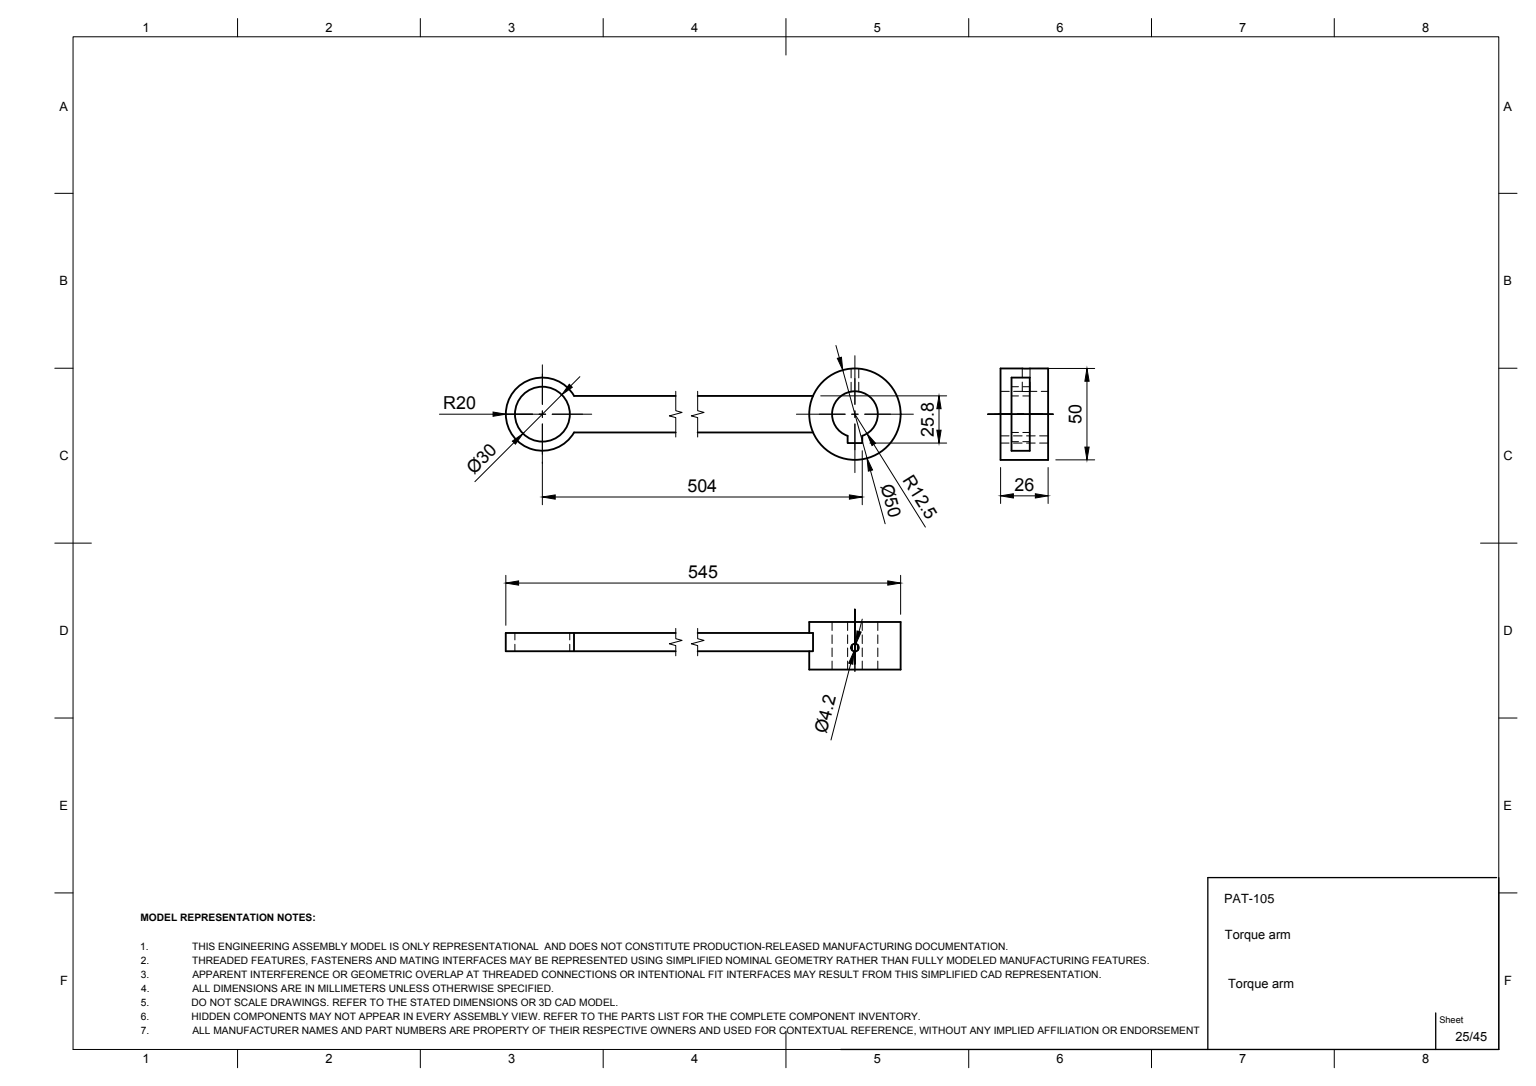
ISO-10303-21;
HEADER;
/* Generated by software containing ST-Developer
 * from STEP Tools, Inc. (www.steptools.com) 
 */

FILE_DESCRIPTION(
/* description */ ('Torque wrench calibration arm'),
/* implementation_level */ '2;1');

FILE_NAME(
/* name */ 'Torque arm.step',
/* time_stamp */ '2026-10-28T03:24:52-07:00',
/* author */ (''),
/* organization */ (''),
/* preprocessor_version */ 'ST-DEVELOPER v20.2',
/* originating_system */ 'Autodesk Translation Framework v15.17.0.0',
/* authorisation */ '');

FILE_SCHEMA (('AUTOMOTIVE_DESIGN { 1 0 10303 214 3 1 1 }'));
ENDSEC;

DATA;
#10=MECHANICAL_DESIGN_GEOMETRIC_PRESENTATION_REPRESENTATION('',(#453),#12783);
#271=B_SPLINE_CURVE_WITH_KNOTS('',3,(#11550,#11551,#11552,#11553,#11554,
#11555,#11556,#11557,#11558,#11559,#11560,#11561,#11562,#11563),
 .UNSPECIFIED.,.F.,.F.,(4,2,2,2,2,2,4),(0.779149138325153,0.792661737650616,
0.871926599437981,0.951191461225347,1.03045632301271,1.10972118480008,1.12323378412554),
 .UNSPECIFIED.);
#272=B_SPLINE_CURVE_WITH_KNOTS('',3,(#11569,#11570,#11571,#11572,#11573,
#11574,#11575,#11576,#11577,#11578,#11579,#11580,#11581,#11582,#11583,#11584,
#11585,#11586),.UNSPECIFIED.,.F.,.F.,(4,2,2,2,2,2,2,2,4),(0.,0.0791442954208927,
0.158288590841785,0.23743275251224,0.316576914182695,0.39572107585315,0.474865237523604,
0.554009532944497,0.63315382836539),.UNSPECIFIED.);
#273=B_SPLINE_CURVE_WITH_KNOTS('',3,(#11587,#11588,#11589,#11590,#11591,
#11592,#11593,#11594,#11595,#11596,#11597,#11598,#11599,#11600,#11601,#11602,
#11603,#11604),.UNSPECIFIED.,.F.,.F.,(4,2,2,2,2,2,2,2,4),(0.63315382836539,
0.712298123786282,0.791442419207175,0.87058658087763,0.949730742548085,
1.02887490421854,1.10801906588899,1.18716336130989,1.26630765673078),
 .UNSPECIFIED.);
#274=B_SPLINE_CURVE_WITH_KNOTS('',3,(#11607,#11608,#11609,#11610,#11611,
#11612,#11613,#11614,#11615,#11616,#11617,#11618,#11619,#11620),
 .UNSPECIFIED.,.F.,.F.,(4,2,2,2,2,2,4),(0.145021497508257,0.158534096833718,
0.237798958621084,0.317063820408449,0.396328682195814,0.47559354398318,
0.489106143308642),.UNSPECIFIED.);
#370=SHAPE_REPRESENTATION_RELATIONSHIP('SRR','None',#12953,#407);
#407=ADVANCED_BREP_SHAPE_REPRESENTATION('',(#505),#12762);
#453=STYLED_ITEM('',(#13205),#505);
#505=MANIFOLD_SOLID_BREP('Body1',#6524);
#608=FACE_BOUND('',#1588,.T.);
#609=FACE_BOUND('',#1590,.T.);
#610=FACE_BOUND('',#1594,.T.);
#611=FACE_BOUND('',#1597,.T.);
#612=FACE_BOUND('',#1600,.T.);
#613=FACE_BOUND('',#1601,.T.);
#614=FACE_BOUND('',#1603,.T.);
#785=PLANE('',#7454);
#786=PLANE('',#7459);
#787=PLANE('',#7460);
#788=PLANE('',#7461);
#789=PLANE('',#7462);
#790=PLANE('',#7463);
#791=PLANE('',#7474);
#792=PLANE('',#7476);
#793=PLANE('',#7477);
#794=PLANE('',#7479);
#795=PLANE('',#7482);
#1109=FACE_OUTER_BOUND('',#1581,.T.);
#1110=FACE_OUTER_BOUND('',#1582,.T.);
#1111=FACE_OUTER_BOUND('',#1583,.T.);
#1112=FACE_OUTER_BOUND('',#1584,.T.);
#1113=FACE_OUTER_BOUND('',#1585,.T.);
#1114=FACE_OUTER_BOUND('',#1586,.T.);
#1115=FACE_OUTER_BOUND('',#1587,.T.);
#1116=FACE_OUTER_BOUND('',#1589,.T.);
#1117=FACE_OUTER_BOUND('',#1591,.T.);
#1118=FACE_OUTER_BOUND('',#1592,.T.);
#1119=FACE_OUTER_BOUND('',#1593,.T.);
#1120=FACE_OUTER_BOUND('',#1595,.T.);
#1121=FACE_OUTER_BOUND('',#1596,.T.);
#1122=FACE_OUTER_BOUND('',#1598,.T.);
#1123=FACE_OUTER_BOUND('',#1599,.T.);
#1124=FACE_OUTER_BOUND('',#1602,.T.);
#1581=EDGE_LOOP('',(#5345,#5346));
#1582=EDGE_LOOP('',(#5347,#5348,#5349,#5350,#5351,#5352,#5353,#5354,#5355));
#1583=EDGE_LOOP('',(#5356,#5357,#5358));
#1584=EDGE_LOOP('',(#5359,#5360,#5361,#5362));
#1585=EDGE_LOOP('',(#5363,#5364,#5365,#5366));
#1586=EDGE_LOOP('',(#5367,#5368,#5369,#5370));
#1587=EDGE_LOOP('',(#5371));
#1588=EDGE_LOOP('',(#5372,#5373,#5374,#5375));
#1589=EDGE_LOOP('',(#5376,#5377,#5378,#5379));
#1590=EDGE_LOOP('',(#5380,#5381,#5382,#5383));
#1591=EDGE_LOOP('',(#5384,#5385,#5386,#5387));
#1592=EDGE_LOOP('',(#5388,#5389,#5390,#5391));
#1593=EDGE_LOOP('',(#5392,#5393,#5394,#5395));
#1594=EDGE_LOOP('',(#5396));
#1595=EDGE_LOOP('',(#5397,#5398,#5399,#5400));
#1596=EDGE_LOOP('',(#5401,#5402,#5403,#5404));
#1597=EDGE_LOOP('',(#5405));
#1598=EDGE_LOOP('',(#5406,#5407,#5408,#5409));
#1599=EDGE_LOOP('',(#5410,#5411,#5412,#5413));
#1600=EDGE_LOOP('',(#5414,#5415));
#1601=EDGE_LOOP('',(#5416,#5417,#5418,#5419));
#1602=EDGE_LOOP('',(#5420));
#1603=EDGE_LOOP('',(#5421,#5422,#5423,#5424));
#2046=LINE('',#11546,#2461);
#2047=LINE('',#11567,#2462);
#2048=LINE('',#11622,#2463);
#2049=LINE('',#11626,#2464);
#2050=LINE('',#11628,#2465);
#2051=LINE('',#11630,#2466);
#2052=LINE('',#11631,#2467);
#2053=LINE('',#11634,#2468);
#2054=LINE('',#11636,#2469);
#2055=LINE('',#11637,#2470);
#2056=LINE('',#11640,#2471);
#2057=LINE('',#11642,#2472);
#2058=LINE('',#11643,#2473);
#2059=LINE('',#11654,#2474);
#2060=LINE('',#11659,#2475);
#2061=LINE('',#11663,#2476);
#2062=LINE('',#11667,#2477);
#2063=LINE('',#11670,#2478);
#2064=LINE('',#11673,#2479);
#2065=LINE('',#11674,#2480);
#2066=LINE('',#11677,#2481);
#2067=LINE('',#11680,#2482);
#2068=LINE('',#11683,#2483);
#2461=VECTOR('',#9060,1.);
#2462=VECTOR('',#9067,0.21);
#2463=VECTOR('',#9072,1.);
#2464=VECTOR('',#9075,1.);
#2465=VECTOR('',#9076,1.);
#2466=VECTOR('',#9077,1.);
#2467=VECTOR('',#9078,1.);
#2468=VECTOR('',#9081,1.);
#2469=VECTOR('',#9082,1.);
#2470=VECTOR('',#9083,1.);
#2471=VECTOR('',#9086,1.);
#2472=VECTOR('',#9087,1.);
#2473=VECTOR('',#9088,1.);
#2474=VECTOR('',#9103,1.5);
#2475=VECTOR('',#9108,1.);
#2476=VECTOR('',#9111,1.);
#2477=VECTOR('',#9116,1.);
#2478=VECTOR('',#9119,1.);
#2479=VECTOR('',#9122,1.);
#2480=VECTOR('',#9123,1.);
#2481=VECTOR('',#9126,1.);
#2482=VECTOR('',#9131,1.);
#2483=VECTOR('',#9134,2.5);
#2827=CIRCLE('',#7455,0.21);
#2828=CIRCLE('',#7457,0.21);
#2829=CIRCLE('',#7458,0.21);
#2830=CIRCLE('',#7464,2.5);
#2831=CIRCLE('',#7465,1.25);
#2832=CIRCLE('',#7467,1.25);
#2833=CIRCLE('',#7469,1.5);
#2834=CIRCLE('',#7470,1.5);
#2835=CIRCLE('',#7472,2.);
#2836=CIRCLE('',#7473,2.);
#2837=CIRCLE('',#7475,2.5);
#2838=CIRCLE('',#7478,2.5);
#2839=CIRCLE('',#7481,2.5);
#3311=VERTEX_POINT('',#11544);
#3312=VERTEX_POINT('',#11545);
#3313=VERTEX_POINT('',#11549);
#3314=VERTEX_POINT('',#11564);
#3315=VERTEX_POINT('',#11566);
#3316=VERTEX_POINT('',#11568);
#3317=VERTEX_POINT('',#11605);
#3318=VERTEX_POINT('',#11624);
#3319=VERTEX_POINT('',#11625);
#3320=VERTEX_POINT('',#11627);
#3321=VERTEX_POINT('',#11629);
#3322=VERTEX_POINT('',#11633);
#3323=VERTEX_POINT('',#11635);
#3324=VERTEX_POINT('',#11639);
#3325=VERTEX_POINT('',#11641);
#3326=VERTEX_POINT('',#11645);
#3327=VERTEX_POINT('',#11651);
#3328=VERTEX_POINT('',#11653);
#3329=VERTEX_POINT('',#11657);
#3330=VERTEX_POINT('',#11658);
#3331=VERTEX_POINT('',#11660);
#3332=VERTEX_POINT('',#11662);
#3333=VERTEX_POINT('',#11666);
#3334=VERTEX_POINT('',#11668);
#3335=VERTEX_POINT('',#11672);
#3336=VERTEX_POINT('',#11676);
#3337=VERTEX_POINT('',#11682);
#4030=EDGE_CURVE('',#3311,#3312,#2046,.T.);
#4031=EDGE_CURVE('',#3311,#3312,#2827,.T.);
#4032=EDGE_CURVE('',#3313,#3311,#271,.T.);
#4033=EDGE_CURVE('',#3314,#3313,#2828,.T.);
#4034=EDGE_CURVE('',#3314,#3315,#2047,.T.);
#4035=EDGE_CURVE('',#3316,#3315,#272,.T.);
#4036=EDGE_CURVE('',#3315,#3316,#273,.T.);
#4037=EDGE_CURVE('',#3317,#3314,#2829,.T.);
#4038=EDGE_CURVE('',#3312,#3317,#274,.T.);
#4039=EDGE_CURVE('',#3317,#3313,#2048,.T.);
#4040=EDGE_CURVE('',#3318,#3319,#2049,.T.);
#4041=EDGE_CURVE('',#3318,#3320,#2050,.T.);
#4042=EDGE_CURVE('',#3321,#3320,#2051,.T.);
#4043=EDGE_CURVE('',#3319,#3321,#2052,.T.);
#4044=EDGE_CURVE('',#3322,#3318,#2053,.T.);
#4045=EDGE_CURVE('',#3322,#3323,#2054,.T.);
#4046=EDGE_CURVE('',#3320,#3323,#2055,.T.);
#4047=EDGE_CURVE('',#3324,#3322,#2056,.T.);
#4048=EDGE_CURVE('',#3325,#3324,#2057,.T.);
#4049=EDGE_CURVE('',#3323,#3325,#2058,.T.);
#4050=EDGE_CURVE('',#3326,#3326,#2830,.T.);
#4051=EDGE_CURVE('',#3325,#3321,#2831,.T.);
#4052=EDGE_CURVE('',#3324,#3319,#2832,.T.);
#4053=EDGE_CURVE('',#3327,#3327,#2833,.T.);
#4054=EDGE_CURVE('',#3327,#3328,#2059,.T.);
#4055=EDGE_CURVE('',#3328,#3328,#2834,.T.);
#4056=EDGE_CURVE('',#3329,#3330,#2060,.T.);
#4057=EDGE_CURVE('',#3331,#3329,#2835,.T.);
#4058=EDGE_CURVE('',#3332,#3331,#2061,.T.);
#4059=EDGE_CURVE('',#3332,#3330,#2836,.T.);
#4060=EDGE_CURVE('',#3332,#3333,#2062,.T.);
#4061=EDGE_CURVE('',#3334,#3333,#2837,.T.);
#4062=EDGE_CURVE('',#3334,#3330,#2063,.T.);
#4063=EDGE_CURVE('',#3335,#3331,#2064,.T.);
#4064=EDGE_CURVE('',#3333,#3335,#2065,.T.);
#4065=EDGE_CURVE('',#3329,#3336,#2066,.T.);
#4066=EDGE_CURVE('',#3335,#3336,#2838,.T.);
#4067=EDGE_CURVE('',#3336,#3334,#2067,.T.);
#4068=EDGE_CURVE('',#3326,#3337,#2068,.T.);
#4069=EDGE_CURVE('',#3337,#3337,#2839,.T.);
#5345=ORIENTED_EDGE('',*,*,#4030,.F.);
#5346=ORIENTED_EDGE('',*,*,#4031,.T.);
#5347=ORIENTED_EDGE('',*,*,#4032,.F.);
#5348=ORIENTED_EDGE('',*,*,#4033,.F.);
#5349=ORIENTED_EDGE('',*,*,#4034,.T.);
#5350=ORIENTED_EDGE('',*,*,#4035,.F.);
#5351=ORIENTED_EDGE('',*,*,#4036,.F.);
#5352=ORIENTED_EDGE('',*,*,#4034,.F.);
#5353=ORIENTED_EDGE('',*,*,#4037,.F.);
#5354=ORIENTED_EDGE('',*,*,#4038,.F.);
#5355=ORIENTED_EDGE('',*,*,#4031,.F.);
#5356=ORIENTED_EDGE('',*,*,#4039,.F.);
#5357=ORIENTED_EDGE('',*,*,#4037,.T.);
#5358=ORIENTED_EDGE('',*,*,#4033,.T.);
#5359=ORIENTED_EDGE('',*,*,#4040,.F.);
#5360=ORIENTED_EDGE('',*,*,#4041,.T.);
#5361=ORIENTED_EDGE('',*,*,#4042,.F.);
#5362=ORIENTED_EDGE('',*,*,#4043,.F.);
#5363=ORIENTED_EDGE('',*,*,#4044,.F.);
#5364=ORIENTED_EDGE('',*,*,#4045,.T.);
#5365=ORIENTED_EDGE('',*,*,#4046,.F.);
#5366=ORIENTED_EDGE('',*,*,#4041,.F.);
#5367=ORIENTED_EDGE('',*,*,#4047,.F.);
#5368=ORIENTED_EDGE('',*,*,#4048,.F.);
#5369=ORIENTED_EDGE('',*,*,#4049,.F.);
#5370=ORIENTED_EDGE('',*,*,#4045,.F.);
#5371=ORIENTED_EDGE('',*,*,#4050,.T.);
#5372=ORIENTED_EDGE('',*,*,#4042,.T.);
#5373=ORIENTED_EDGE('',*,*,#4046,.T.);
#5374=ORIENTED_EDGE('',*,*,#4049,.T.);
#5375=ORIENTED_EDGE('',*,*,#4051,.T.);
#5376=ORIENTED_EDGE('',*,*,#4043,.T.);
#5377=ORIENTED_EDGE('',*,*,#4051,.F.);
#5378=ORIENTED_EDGE('',*,*,#4048,.T.);
#5379=ORIENTED_EDGE('',*,*,#4052,.T.);
#5380=ORIENTED_EDGE('',*,*,#4038,.T.);
#5381=ORIENTED_EDGE('',*,*,#4039,.T.);
#5382=ORIENTED_EDGE('',*,*,#4032,.T.);
#5383=ORIENTED_EDGE('',*,*,#4030,.T.);
#5384=ORIENTED_EDGE('',*,*,#4053,.F.);
#5385=ORIENTED_EDGE('',*,*,#4054,.T.);
#5386=ORIENTED_EDGE('',*,*,#4055,.F.);
#5387=ORIENTED_EDGE('',*,*,#4054,.F.);
#5388=ORIENTED_EDGE('',*,*,#4056,.F.);
#5389=ORIENTED_EDGE('',*,*,#4057,.F.);
#5390=ORIENTED_EDGE('',*,*,#4058,.F.);
#5391=ORIENTED_EDGE('',*,*,#4059,.T.);
#5392=ORIENTED_EDGE('',*,*,#4059,.F.);
#5393=ORIENTED_EDGE('',*,*,#4060,.T.);
#5394=ORIENTED_EDGE('',*,*,#4061,.F.);
#5395=ORIENTED_EDGE('',*,*,#4062,.T.);
#5396=ORIENTED_EDGE('',*,*,#4053,.T.);
#5397=ORIENTED_EDGE('',*,*,#4058,.T.);
#5398=ORIENTED_EDGE('',*,*,#4063,.F.);
#5399=ORIENTED_EDGE('',*,*,#4064,.F.);
#5400=ORIENTED_EDGE('',*,*,#4060,.F.);
#5401=ORIENTED_EDGE('',*,*,#4065,.T.);
#5402=ORIENTED_EDGE('',*,*,#4066,.F.);
#5403=ORIENTED_EDGE('',*,*,#4063,.T.);
#5404=ORIENTED_EDGE('',*,*,#4057,.T.);
#5405=ORIENTED_EDGE('',*,*,#4055,.T.);
#5406=ORIENTED_EDGE('',*,*,#4056,.T.);
#5407=ORIENTED_EDGE('',*,*,#4062,.F.);
#5408=ORIENTED_EDGE('',*,*,#4067,.F.);
#5409=ORIENTED_EDGE('',*,*,#4065,.F.);
#5410=ORIENTED_EDGE('',*,*,#4050,.F.);
#5411=ORIENTED_EDGE('',*,*,#4068,.T.);
#5412=ORIENTED_EDGE('',*,*,#4069,.T.);
#5413=ORIENTED_EDGE('',*,*,#4068,.F.);
#5414=ORIENTED_EDGE('',*,*,#4035,.T.);
#5415=ORIENTED_EDGE('',*,*,#4036,.T.);
#5416=ORIENTED_EDGE('',*,*,#4064,.T.);
#5417=ORIENTED_EDGE('',*,*,#4066,.T.);
#5418=ORIENTED_EDGE('',*,*,#4067,.T.);
#5419=ORIENTED_EDGE('',*,*,#4061,.T.);
#5420=ORIENTED_EDGE('',*,*,#4069,.F.);
#5421=ORIENTED_EDGE('',*,*,#4040,.T.);
#5422=ORIENTED_EDGE('',*,*,#4052,.F.);
#5423=ORIENTED_EDGE('',*,*,#4047,.T.);
#5424=ORIENTED_EDGE('',*,*,#4044,.T.);
#6056=CYLINDRICAL_SURFACE('',#7456,0.21);
#6057=CYLINDRICAL_SURFACE('',#7466,1.25);
#6058=CYLINDRICAL_SURFACE('',#7468,1.5);
#6059=CYLINDRICAL_SURFACE('',#7471,2.);
#6060=CYLINDRICAL_SURFACE('',#7480,2.5);
#6334=ADVANCED_FACE('',(#1109),#785,.T.);
#6335=ADVANCED_FACE('',(#1110),#6056,.F.);
#6336=ADVANCED_FACE('',(#1111),#786,.T.);
#6337=ADVANCED_FACE('',(#1112),#787,.F.);
#6338=ADVANCED_FACE('',(#1113),#788,.F.);
#6339=ADVANCED_FACE('',(#1114),#789,.F.);
#6340=ADVANCED_FACE('',(#1115,#608),#790,.T.);
#6341=ADVANCED_FACE('',(#1116,#609),#6057,.F.);
#6342=ADVANCED_FACE('',(#1117),#6058,.F.);
#6343=ADVANCED_FACE('',(#1118),#6059,.T.);
#6344=ADVANCED_FACE('',(#1119,#610),#791,.F.);
#6345=ADVANCED_FACE('',(#1120),#792,.T.);
#6346=ADVANCED_FACE('',(#1121,#611),#793,.T.);
#6347=ADVANCED_FACE('',(#1122),#794,.T.);
#6348=ADVANCED_FACE('',(#1123,#612,#613),#6060,.T.);
#6349=ADVANCED_FACE('',(#1124,#614),#795,.F.);
#6524=CLOSED_SHELL('',(#6334,#6335,#6336,#6337,#6338,#6339,#6340,#6341,
#6342,#6343,#6344,#6345,#6346,#6347,#6348,#6349));
#7453=AXIS2_PLACEMENT_3D('',#11542,#9056,#9057);
#7454=AXIS2_PLACEMENT_3D('',#11543,#9058,#9059);
#7455=AXIS2_PLACEMENT_3D('',#11547,#9061,#9062);
#7456=AXIS2_PLACEMENT_3D('',#11548,#9063,#9064);
#7457=AXIS2_PLACEMENT_3D('',#11565,#9065,#9066);
#7458=AXIS2_PLACEMENT_3D('',#11606,#9068,#9069);
#7459=AXIS2_PLACEMENT_3D('',#11621,#9070,#9071);
#7460=AXIS2_PLACEMENT_3D('',#11623,#9073,#9074);
#7461=AXIS2_PLACEMENT_3D('',#11632,#9079,#9080);
#7462=AXIS2_PLACEMENT_3D('',#11638,#9084,#9085);
#7463=AXIS2_PLACEMENT_3D('',#11644,#9089,#9090);
#7464=AXIS2_PLACEMENT_3D('',#11646,#9091,#9092);
#7465=AXIS2_PLACEMENT_3D('',#11647,#9093,#9094);
#7466=AXIS2_PLACEMENT_3D('',#11648,#9095,#9096);
#7467=AXIS2_PLACEMENT_3D('',#11649,#9097,#9098);
#7468=AXIS2_PLACEMENT_3D('',#11650,#9099,#9100);
#7469=AXIS2_PLACEMENT_3D('',#11652,#9101,#9102);
#7470=AXIS2_PLACEMENT_3D('',#11655,#9104,#9105);
#7471=AXIS2_PLACEMENT_3D('',#11656,#9106,#9107);
#7472=AXIS2_PLACEMENT_3D('',#11661,#9109,#9110);
#7473=AXIS2_PLACEMENT_3D('',#11664,#9112,#9113);
#7474=AXIS2_PLACEMENT_3D('',#11665,#9114,#9115);
#7475=AXIS2_PLACEMENT_3D('',#11669,#9117,#9118);
#7476=AXIS2_PLACEMENT_3D('',#11671,#9120,#9121);
#7477=AXIS2_PLACEMENT_3D('',#11675,#9124,#9125);
#7478=AXIS2_PLACEMENT_3D('',#11678,#9127,#9128);
#7479=AXIS2_PLACEMENT_3D('',#11679,#9129,#9130);
#7480=AXIS2_PLACEMENT_3D('',#11681,#9132,#9133);
#7481=AXIS2_PLACEMENT_3D('',#11684,#9135,#9136);
#7482=AXIS2_PLACEMENT_3D('',#11685,#9137,#9138);
#9056=DIRECTION('axis',(0.,0.,1.));
#9057=DIRECTION('refdir',(1.,0.,0.));
#9058=DIRECTION('center_axis',(0.,0.,1.));
#9059=DIRECTION('ref_axis',(1.,0.,0.));
#9060=DIRECTION('',(0.,1.,0.));
#9061=DIRECTION('center_axis',(0.,0.,1.));
#9062=DIRECTION('ref_axis',(1.,0.,0.));
#9063=DIRECTION('center_axis',(0.,0.,1.));
#9064=DIRECTION('ref_axis',(1.,0.,0.));
#9065=DIRECTION('center_axis',(0.,0.,1.));
#9066=DIRECTION('ref_axis',(1.,0.,0.));
#9067=DIRECTION('',(0.,0.,1.));
#9068=DIRECTION('center_axis',(0.,0.,1.));
#9069=DIRECTION('ref_axis',(1.,0.,0.));
#9070=DIRECTION('center_axis',(0.,0.,1.));
#9071=DIRECTION('ref_axis',(1.,0.,0.));
#9072=DIRECTION('',(0.,-1.,0.));
#9073=DIRECTION('center_axis',(-1.,0.,0.));
#9074=DIRECTION('ref_axis',(0.,0.,1.));
#9075=DIRECTION('',(0.,0.,1.));
#9076=DIRECTION('',(0.,1.,0.));
#9077=DIRECTION('',(0.,0.,-1.));
#9078=DIRECTION('',(0.,1.,0.));
#9079=DIRECTION('center_axis',(0.,0.,-1.));
#9080=DIRECTION('ref_axis',(-1.,0.,0.));
#9081=DIRECTION('',(-1.,0.,0.));
#9082=DIRECTION('',(0.,1.,0.));
#9083=DIRECTION('',(1.,0.,0.));
#9084=DIRECTION('center_axis',(1.,0.,0.));
#9085=DIRECTION('ref_axis',(0.,0.,-1.));
#9086=DIRECTION('',(0.,0.,-1.));
#9087=DIRECTION('',(0.,-1.,0.));
#9088=DIRECTION('',(0.,0.,1.));
#9089=DIRECTION('center_axis',(0.,1.,0.));
#9090=DIRECTION('ref_axis',(1.,0.,0.));
#9091=DIRECTION('center_axis',(0.,1.,0.));
#9092=DIRECTION('ref_axis',(1.,0.,0.));
#9093=DIRECTION('center_axis',(0.,-1.,0.));
#9094=DIRECTION('ref_axis',(1.,0.,0.));
#9095=DIRECTION('center_axis',(0.,1.,0.));
#9096=DIRECTION('ref_axis',(-1.83697019872103E-16,0.,1.));
#9097=DIRECTION('center_axis',(0.,-1.,0.));
#9098=DIRECTION('ref_axis',(1.,0.,0.));
#9099=DIRECTION('center_axis',(0.,1.,0.));
#9100=DIRECTION('ref_axis',(1.,0.,0.));
#9101=DIRECTION('center_axis',(0.,1.,0.));
#9102=DIRECTION('ref_axis',(1.,0.,0.));
#9103=DIRECTION('',(0.,1.,0.));
#9104=DIRECTION('center_axis',(0.,-1.,0.));
#9105=DIRECTION('ref_axis',(1.,0.,0.));
#9106=DIRECTION('center_axis',(0.,1.,0.));
#9107=DIRECTION('ref_axis',(1.,0.,0.));
#9108=DIRECTION('',(0.,-1.,0.));
#9109=DIRECTION('center_axis',(0.,1.,0.));
#9110=DIRECTION('ref_axis',(1.,0.,0.));
#9111=DIRECTION('',(0.,1.,0.));
#9112=DIRECTION('center_axis',(0.,1.,0.));
#9113=DIRECTION('ref_axis',(1.,0.,0.));
#9114=DIRECTION('center_axis',(0.,1.,0.));
#9115=DIRECTION('ref_axis',(1.,0.,0.));
#9116=DIRECTION('',(-1.,0.,0.));
#9117=DIRECTION('center_axis',(0.,-1.,0.));
#9118=DIRECTION('ref_axis',(1.,0.,0.));
#9119=DIRECTION('',(1.,0.,0.));
#9120=DIRECTION('center_axis',(0.,0.,1.));
#9121=DIRECTION('ref_axis',(1.,0.,0.));
#9122=DIRECTION('',(1.,0.,0.));
#9123=DIRECTION('',(0.,1.,0.));
#9124=DIRECTION('center_axis',(0.,1.,0.));
#9125=DIRECTION('ref_axis',(0.,0.,1.));
#9126=DIRECTION('',(-1.,0.,0.));
#9127=DIRECTION('center_axis',(0.,1.,0.));
#9128=DIRECTION('ref_axis',(1.,0.,0.));
#9129=DIRECTION('center_axis',(0.,0.,-1.));
#9130=DIRECTION('ref_axis',(-1.,0.,0.));
#9131=DIRECTION('',(0.,-1.,0.));
#9132=DIRECTION('center_axis',(0.,1.,0.));
#9133=DIRECTION('ref_axis',(1.,0.,0.));
#9134=DIRECTION('',(0.,-1.,0.));
#9135=DIRECTION('center_axis',(0.,1.,0.));
#9136=DIRECTION('ref_axis',(1.,0.,0.));
#9137=DIRECTION('center_axis',(0.,1.,0.));
#9138=DIRECTION('ref_axis',(1.,0.,0.));
#11542=CARTESIAN_POINT('',(0.,0.,0.));
#11543=CARTESIAN_POINT('Origin',(0.,8.8,9.24));
#11544=CARTESIAN_POINT('',(0.157797338380593,8.66143593539449,9.24));
#11545=CARTESIAN_POINT('',(0.157797338380593,8.93856406460551,9.24));
#11546=CARTESIAN_POINT('',(0.157797338380593,7.4,9.24));
#11547=CARTESIAN_POINT('Origin',(0.,8.8,9.24));
#11548=CARTESIAN_POINT('Origin',(0.,8.8,9.24));
#11549=CARTESIAN_POINT('',(-0.157797338380593,8.66143593539449,9.24));
#11550=CARTESIAN_POINT('Ctrl Pts',(-0.157797338380593,8.66143593539449,
9.24));
#11551=CARTESIAN_POINT('Ctrl Pts',(-0.154774443077063,8.65799344953455,
9.24038468131702));
#11552=CARTESIAN_POINT('Ctrl Pts',(-0.151666037725851,8.6546811896275,9.24076896680743));
#11553=CARTESIAN_POINT('Ctrl Pts',(-0.129876016991636,8.63289116889329,
9.24337594943507));
#11554=CARTESIAN_POINT('Ctrl Pts',(-0.1062955610194,8.61673756788121,9.24574191032087));
#11555=CARTESIAN_POINT('Ctrl Pts',(-0.054570423856847,8.59529060980459,
9.24907714823024));
#11556=CARTESIAN_POINT('Ctrl Pts',(-0.0264216205957885,8.59,9.25));
#11557=CARTESIAN_POINT('Ctrl Pts',(0.0264216205957884,8.59,9.25));
#11558=CARTESIAN_POINT('Ctrl Pts',(0.054570423856847,8.59529060980459,9.24907714823024));
#11559=CARTESIAN_POINT('Ctrl Pts',(0.1062955610194,8.61673756788121,9.24574191032087));
#11560=CARTESIAN_POINT('Ctrl Pts',(0.129876016991636,8.63289116889329,9.24337594943507));
#11561=CARTESIAN_POINT('Ctrl Pts',(0.151666037725851,8.6546811896275,9.24076896680743));
#11562=CARTESIAN_POINT('Ctrl Pts',(0.154774443077063,8.65799344953455,9.24038468131702));
#11563=CARTESIAN_POINT('Ctrl Pts',(0.157797338380593,8.66143593539449,9.24));
#11564=CARTESIAN_POINT('',(-0.21,8.8,9.24));
#11565=CARTESIAN_POINT('Origin',(0.,8.8,9.24));
#11566=CARTESIAN_POINT('',(-0.21,8.8,10.4911643863864));
#11567=CARTESIAN_POINT('',(-0.21,8.8,9.24));
#11568=CARTESIAN_POINT('',(0.21,8.8,10.4911643863864));
#11569=CARTESIAN_POINT('Ctrl Pts',(0.21,8.8,10.4911643863864));
#11570=CARTESIAN_POINT('Ctrl Pts',(0.21,8.77361856819303,10.4911643863864));
#11571=CARTESIAN_POINT('Ctrl Pts',(0.204725118204866,8.74548720786942,10.4916266149403));
#11572=CARTESIAN_POINT('Ctrl Pts',(0.183289989572642,8.69375124157695,10.4932950771364));
#11573=CARTESIAN_POINT('Ctrl Pts',(0.16713042375487,8.67014557565652,10.4944771047991));
#11574=CARTESIAN_POINT('Ctrl Pts',(0.129854455840894,8.63286960774255,10.4966951003339));
#11575=CARTESIAN_POINT('Ctrl Pts',(0.106248776012194,8.61671001748363,10.4978753058977));
#11576=CARTESIAN_POINT('Ctrl Pts',(0.0545127635959799,8.59527487020396,
10.4995395985687));
#11577=CARTESIAN_POINT('Ctrl Pts',(0.0263813872234849,8.59,10.5));
#11578=CARTESIAN_POINT('Ctrl Pts',(-0.0263813872234849,8.59,10.5));
#11579=CARTESIAN_POINT('Ctrl Pts',(-0.0545127635959799,8.59527487020396,
10.4995395985687));
#11580=CARTESIAN_POINT('Ctrl Pts',(-0.106248776012194,8.61671001748363,
10.4978753058977));
#11581=CARTESIAN_POINT('Ctrl Pts',(-0.129854455840894,8.63286960774255,
10.4966951003339));
#11582=CARTESIAN_POINT('Ctrl Pts',(-0.16713042375487,8.67014557565652,10.4944771047991));
#11583=CARTESIAN_POINT('Ctrl Pts',(-0.183289989572642,8.69375124157695,
10.4932950771364));
#11584=CARTESIAN_POINT('Ctrl Pts',(-0.204725118204866,8.74548720786942,
10.4916266149403));
#11585=CARTESIAN_POINT('Ctrl Pts',(-0.21,8.77361856819304,10.4911643863864));
#11586=CARTESIAN_POINT('Ctrl Pts',(-0.21,8.8,10.4911643863864));
#11587=CARTESIAN_POINT('Ctrl Pts',(-0.21,8.8,10.4911643863864));
#11588=CARTESIAN_POINT('Ctrl Pts',(-0.21,8.82638143180696,10.4911643863864));
#11589=CARTESIAN_POINT('Ctrl Pts',(-0.204725118204866,8.85451279213058,
10.4916266149403));
#11590=CARTESIAN_POINT('Ctrl Pts',(-0.183289989572642,8.90624875842305,
10.4932950771364));
#11591=CARTESIAN_POINT('Ctrl Pts',(-0.16713042375487,8.92985442434348,10.4944771047991));
#11592=CARTESIAN_POINT('Ctrl Pts',(-0.129854455840894,8.96713039225746,
10.4966951003339));
#11593=CARTESIAN_POINT('Ctrl Pts',(-0.106248776012194,8.98328998251637,
10.4978753058977));
#11594=CARTESIAN_POINT('Ctrl Pts',(-0.05451276359598,9.00472512979604,10.4995395985687));
#11595=CARTESIAN_POINT('Ctrl Pts',(-0.026381387223485,9.01,10.5));
#11596=CARTESIAN_POINT('Ctrl Pts',(0.0263813872234849,9.01,10.5));
#11597=CARTESIAN_POINT('Ctrl Pts',(0.0545127635959799,9.00472512979604,
10.4995395985687));
#11598=CARTESIAN_POINT('Ctrl Pts',(0.106248776012194,8.98328998251637,10.4978753058977));
#11599=CARTESIAN_POINT('Ctrl Pts',(0.129854455840894,8.96713039225746,10.4966951003339));
#11600=CARTESIAN_POINT('Ctrl Pts',(0.16713042375487,8.92985442434348,10.4944771047991));
#11601=CARTESIAN_POINT('Ctrl Pts',(0.183289989572642,8.90624875842305,10.4932950771364));
#11602=CARTESIAN_POINT('Ctrl Pts',(0.204725118204866,8.85451279213058,10.4916266149403));
#11603=CARTESIAN_POINT('Ctrl Pts',(0.21,8.82638143180697,10.4911643863864));
#11604=CARTESIAN_POINT('Ctrl Pts',(0.21,8.8,10.4911643863864));
#11605=CARTESIAN_POINT('',(-0.157797338380593,8.93856406460551,9.24));
#11606=CARTESIAN_POINT('Origin',(0.,8.8,9.24));
#11607=CARTESIAN_POINT('Ctrl Pts',(0.157797338380593,8.93856406460551,9.24));
#11608=CARTESIAN_POINT('Ctrl Pts',(0.154774443077063,8.94200655046545,9.24038468131702));
#11609=CARTESIAN_POINT('Ctrl Pts',(0.151666037725851,8.9453188103725,9.24076896680743));
#11610=CARTESIAN_POINT('Ctrl Pts',(0.129876016991636,8.96710883110671,9.24337594943507));
#11611=CARTESIAN_POINT('Ctrl Pts',(0.1062955610194,8.98326243211879,9.24574191032087));
#11612=CARTESIAN_POINT('Ctrl Pts',(0.054570423856847,9.00470939019541,9.24907714823024));
#11613=CARTESIAN_POINT('Ctrl Pts',(0.0264216205957885,9.01,9.25));
#11614=CARTESIAN_POINT('Ctrl Pts',(-0.0264216205957884,9.01,9.25));
#11615=CARTESIAN_POINT('Ctrl Pts',(-0.054570423856847,9.00470939019541,
9.24907714823024));
#11616=CARTESIAN_POINT('Ctrl Pts',(-0.1062955610194,8.98326243211879,9.24574191032087));
#11617=CARTESIAN_POINT('Ctrl Pts',(-0.129876016991636,8.96710883110671,
9.24337594943507));
#11618=CARTESIAN_POINT('Ctrl Pts',(-0.151666037725851,8.9453188103725,9.24076896680743));
#11619=CARTESIAN_POINT('Ctrl Pts',(-0.154774443077063,8.94200655046545,
9.24038468131702));
#11620=CARTESIAN_POINT('Ctrl Pts',(-0.157797338380593,8.93856406460551,
9.24));
#11621=CARTESIAN_POINT('Origin',(0.,8.8,9.24));
#11622=CARTESIAN_POINT('',(-0.157797338380593,7.4,9.24));
#11623=CARTESIAN_POINT('Origin',(-0.4,7.3,6.42));
#11624=CARTESIAN_POINT('',(-0.4,7.4,6.42));
#11625=CARTESIAN_POINT('',(-0.4,7.4,6.8157280717673));
#11626=CARTESIAN_POINT('',(-0.4,7.4,7.21));
#11627=CARTESIAN_POINT('',(-0.4,10.,6.42));
#11628=CARTESIAN_POINT('',(-0.4,7.3,6.42));
#11629=CARTESIAN_POINT('',(-0.4,10.,6.8157280717673));
#11630=CARTESIAN_POINT('',(-0.4,10.,7.21));
#11631=CARTESIAN_POINT('',(-0.4,7.4,6.8157280717673));
#11632=CARTESIAN_POINT('Origin',(0.4,7.3,6.42));
#11633=CARTESIAN_POINT('',(0.4,7.4,6.42));
#11634=CARTESIAN_POINT('',(0.2,7.4,6.42));
#11635=CARTESIAN_POINT('',(0.4,10.,6.42));
#11636=CARTESIAN_POINT('',(0.4,7.3,6.42));
#11637=CARTESIAN_POINT('',(0.2,10.,6.42));
#11638=CARTESIAN_POINT('Origin',(0.4,7.3,8.));
#11639=CARTESIAN_POINT('',(0.4,7.4,6.8157280717673));
#11640=CARTESIAN_POINT('',(0.4,7.4,8.));
#11641=CARTESIAN_POINT('',(0.4,10.,6.8157280717673));
#11642=CARTESIAN_POINT('',(0.4,7.4,6.8157280717673));
#11643=CARTESIAN_POINT('',(0.4,10.,8.));
#11644=CARTESIAN_POINT('Origin',(0.,10.,8.));
#11645=CARTESIAN_POINT('',(-2.5,10.,8.));
#11646=CARTESIAN_POINT('Origin',(0.,10.,8.));
#11647=CARTESIAN_POINT('Origin',(0.,10.,8.));
#11648=CARTESIAN_POINT('Origin',(0.,7.4,8.));
#11649=CARTESIAN_POINT('Origin',(0.,7.4,8.));
#11650=CARTESIAN_POINT('Origin',(50.,7.9,8.));
#11651=CARTESIAN_POINT('',(48.5,8.,8.));
#11652=CARTESIAN_POINT('Origin',(50.,8.,8.));
#11653=CARTESIAN_POINT('',(48.5,9.,8.));
#11654=CARTESIAN_POINT('',(48.5,7.9,8.));
#11655=CARTESIAN_POINT('Origin',(50.,9.,8.));
#11656=CARTESIAN_POINT('Origin',(50.,8.,8.));
#11657=CARTESIAN_POINT('',(48.2679491924311,9.,7.));
#11658=CARTESIAN_POINT('',(48.2679491924311,8.,7.));
#11659=CARTESIAN_POINT('',(48.2679491924311,8.,7.));
#11660=CARTESIAN_POINT('',(48.2679491924311,9.,9.));
#11661=CARTESIAN_POINT('Origin',(50.,9.,8.));
#11662=CARTESIAN_POINT('',(48.2679491924311,8.,9.));
#11663=CARTESIAN_POINT('',(48.2679491924311,8.,9.));
#11664=CARTESIAN_POINT('Origin',(50.,8.,8.));
#11665=CARTESIAN_POINT('Origin',(25.75,8.,8.));
#11666=CARTESIAN_POINT('',(2.29128784747792,8.,9.));
#11667=CARTESIAN_POINT('',(50.,8.,9.));
#11668=CARTESIAN_POINT('',(2.29128784747792,8.,7.));
#11669=CARTESIAN_POINT('Origin',(0.,8.,8.));
#11670=CARTESIAN_POINT('',(1.5,8.,7.));
#11671=CARTESIAN_POINT('Origin',(1.5,8.,9.));
#11672=CARTESIAN_POINT('',(2.29128784747792,9.,9.));
#11673=CARTESIAN_POINT('',(50.,9.,9.));
#11674=CARTESIAN_POINT('',(2.29128784747792,7.4,9.));
#11675=CARTESIAN_POINT('Origin',(25.75,9.,8.));
#11676=CARTESIAN_POINT('',(2.29128784747792,9.,7.));
#11677=CARTESIAN_POINT('',(1.5,9.,7.));
#11678=CARTESIAN_POINT('Origin',(0.,9.,8.));
#11679=CARTESIAN_POINT('Origin',(50.,8.,7.));
#11680=CARTESIAN_POINT('',(2.29128784747792,7.4,7.));
#11681=CARTESIAN_POINT('Origin',(0.,7.4,8.));
#11682=CARTESIAN_POINT('',(-2.5,7.4,8.));
#11683=CARTESIAN_POINT('',(-2.5,7.4,8.));
#11684=CARTESIAN_POINT('Origin',(0.,7.4,8.));
#11685=CARTESIAN_POINT('Origin',(0.,7.4,8.));
#12718=UNCERTAINTY_MEASURE_WITH_UNIT(LENGTH_MEASURE(0.001),#12784,
'DISTANCE_ACCURACY_VALUE',
'Maximum model space distance between geometric entities at asserted c
onnectivities');
#12739=UNCERTAINTY_MEASURE_WITH_UNIT(LENGTH_MEASURE(0.001),#12784,
'DISTANCE_ACCURACY_VALUE',
'Maximum model space distance between geometric entities at asserted c
onnectivities');
#12762=(
GEOMETRIC_REPRESENTATION_CONTEXT(3)
GLOBAL_UNCERTAINTY_ASSIGNED_CONTEXT((#12718))
GLOBAL_UNIT_ASSIGNED_CONTEXT((#12784,#12786,#12787))
REPRESENTATION_CONTEXT('','3D')
);
#12783=(
GEOMETRIC_REPRESENTATION_CONTEXT(3)
GLOBAL_UNCERTAINTY_ASSIGNED_CONTEXT((#12739))
GLOBAL_UNIT_ASSIGNED_CONTEXT((#12784,#12786,#12787))
REPRESENTATION_CONTEXT('','3D')
);
#12784=(
LENGTH_UNIT()
NAMED_UNIT(*)
SI_UNIT(.CENTI.,.METRE.)
);
#12786=(
NAMED_UNIT(*)
PLANE_ANGLE_UNIT()
SI_UNIT($,.RADIAN.)
);
#12787=(
NAMED_UNIT(*)
SI_UNIT($,.STERADIAN.)
SOLID_ANGLE_UNIT()
);
#12810=SHAPE_DEFINITION_REPRESENTATION(#12879,#12953);
#12879=PRODUCT_DEFINITION_SHAPE('',$,#12997);
#12953=SHAPE_REPRESENTATION('',(#7453),#12762);
#12974=PRODUCT_DEFINITION_CONTEXT('part definition',#13105,'design');
#12997=PRODUCT_DEFINITION('Torque arm','Torque arm',#13040,#12974);
#13040=PRODUCT_DEFINITION_FORMATION('',$,#13129);
#13105=APPLICATION_CONTEXT(
'Core Data for Automotive Mechanical Design Process');
#13106=PRODUCT_CONTEXT('part definition',#13105,'mechanical');
#13129=PRODUCT('Torque arm','Torque arm','Torque arm',(#13106));
#13199=COLOUR_RGB('Sky Blue',0.24,0.69,0.87);
#13200=FILL_AREA_STYLE_COLOUR('',#13199);
#13201=FILL_AREA_STYLE('',(#13200));
#13202=SURFACE_STYLE_FILL_AREA(#13201);
#13203=SURFACE_SIDE_STYLE('',(#13202));
#13204=SURFACE_STYLE_USAGE(.BOTH.,#13203);
#13205=PRESENTATION_STYLE_ASSIGNMENT((#13204));
ENDSEC;
END-ISO-10303-21;
